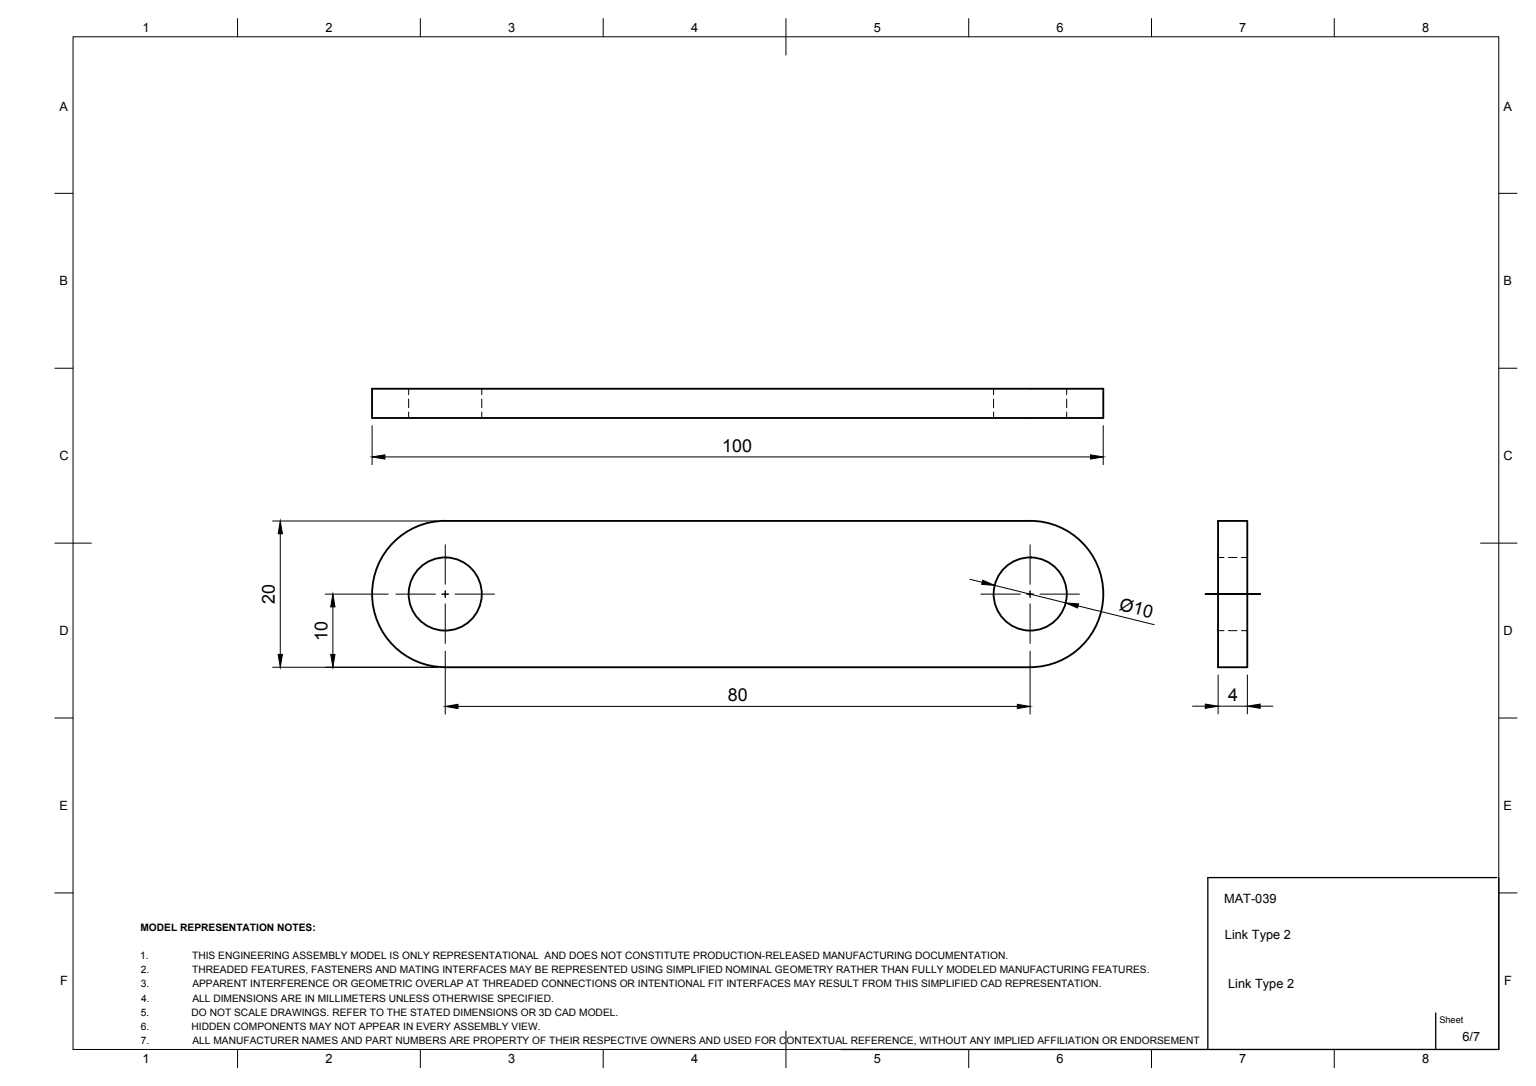
ISO-10303-21;
HEADER;
/* Generated by software containing ST-Developer
 * from STEP Tools, Inc. (www.steptools.com) 
 */

FILE_DESCRIPTION(
/* description */ ('STEP AP214'),
/* implementation_level */ '2;1');

FILE_NAME(
/* name */ 'Link Type 2.step',
/* time_stamp */ '2026-11-14T21:46:24-08:00',
/* author */ (''),
/* organization */ (''),
/* preprocessor_version */ 'ST-DEVELOPER v20.2',
/* originating_system */ 'Autodesk Translation Framework v15.17.0.0',
/* authorisation */ '');

FILE_SCHEMA (('AUTOMOTIVE_DESIGN { 1 0 10303 214 3 1 1 }'));
ENDSEC;

DATA;
#10=MECHANICAL_DESIGN_GEOMETRIC_PRESENTATION_REPRESENTATION('',(#94),#7783);
#80=SHAPE_REPRESENTATION_RELATIONSHIP('SRR','None',#7825,#87);
#87=ADVANCED_BREP_SHAPE_REPRESENTATION('',(#101),#7781);
#94=STYLED_ITEM('',(#7871),#101);
#101=MANIFOLD_SOLID_BREP('Body1',#4169);
#151=FACE_BOUND('',#1584,.T.);
#152=FACE_BOUND('',#1585,.T.);
#153=FACE_BOUND('',#1587,.T.);
#154=FACE_BOUND('',#1588,.T.);
#270=PLANE('',#4656);
#271=PLANE('',#4658);
#272=PLANE('',#4660);
#273=PLANE('',#4662);
#603=LINE('',#7614,#962);
#604=LINE('',#7620,#963);
#605=LINE('',#7627,#964);
#606=LINE('',#7630,#965);
#607=LINE('',#7633,#966);
#608=LINE('',#7636,#967);
#609=LINE('',#7639,#968);
#610=LINE('',#7642,#969);
#611=LINE('',#7644,#970);
#612=LINE('',#7646,#971);
#962=VECTOR('',#5826,5.);
#963=VECTOR('',#5833,5.);
#964=VECTOR('',#5840,1000.);
#965=VECTOR('',#5843,1000.);
#966=VECTOR('',#5846,1000.);
#967=VECTOR('',#5849,1000.);
#968=VECTOR('',#5852,1000.);
#969=VECTOR('',#5855,1000.);
#970=VECTOR('',#5858,1000.);
#971=VECTOR('',#5861,1000.);
#1078=CYLINDRICAL_SURFACE('',#4647,5.);
#1079=CYLINDRICAL_SURFACE('',#4650,5.);
#1080=CYLINDRICAL_SURFACE('',#4653,10.);
#1081=CYLINDRICAL_SURFACE('',#4661,10.);
#1298=FACE_OUTER_BOUND('',#1580,.T.);
#1299=FACE_OUTER_BOUND('',#1581,.T.);
#1300=FACE_OUTER_BOUND('',#1582,.T.);
#1301=FACE_OUTER_BOUND('',#1583,.T.);
#1302=FACE_OUTER_BOUND('',#1586,.T.);
#1303=FACE_OUTER_BOUND('',#1589,.T.);
#1304=FACE_OUTER_BOUND('',#1590,.T.);
#1305=FACE_OUTER_BOUND('',#1591,.T.);
#1580=EDGE_LOOP('',(#3768,#3769,#3770,#3771));
#1581=EDGE_LOOP('',(#3772,#3773,#3774,#3775));
#1582=EDGE_LOOP('',(#3776,#3777,#3778,#3779));
#1583=EDGE_LOOP('',(#3780,#3781,#3782,#3783));
#1584=EDGE_LOOP('',(#3784));
#1585=EDGE_LOOP('',(#3785));
#1586=EDGE_LOOP('',(#3786,#3787,#3788,#3789));
#1587=EDGE_LOOP('',(#3790));
#1588=EDGE_LOOP('',(#3791));
#1589=EDGE_LOOP('',(#3792,#3793,#3794,#3795));
#1590=EDGE_LOOP('',(#3796,#3797,#3798,#3799));
#1591=EDGE_LOOP('',(#3800,#3801,#3802,#3803));
#1800=CIRCLE('',#4648,5.);
#1801=CIRCLE('',#4649,5.);
#1802=CIRCLE('',#4651,5.);
#1803=CIRCLE('',#4652,5.);
#1804=CIRCLE('',#4654,10.);
#1805=CIRCLE('',#4655,10.);
#1806=CIRCLE('',#4657,10.);
#1807=CIRCLE('',#4659,10.);
#2142=VERTEX_POINT('',#7611);
#2143=VERTEX_POINT('',#7613);
#2144=VERTEX_POINT('',#7617);
#2145=VERTEX_POINT('',#7619);
#2146=VERTEX_POINT('',#7623);
#2147=VERTEX_POINT('',#7624);
#2148=VERTEX_POINT('',#7626);
#2149=VERTEX_POINT('',#7628);
#2150=VERTEX_POINT('',#7632);
#2151=VERTEX_POINT('',#7634);
#2152=VERTEX_POINT('',#7638);
#2153=VERTEX_POINT('',#7640);
#2691=EDGE_CURVE('',#2142,#2142,#1800,.T.);
#2692=EDGE_CURVE('',#2142,#2143,#603,.T.);
#2693=EDGE_CURVE('',#2143,#2143,#1801,.T.);
#2694=EDGE_CURVE('',#2144,#2144,#1802,.T.);
#2695=EDGE_CURVE('',#2144,#2145,#604,.T.);
#2696=EDGE_CURVE('',#2145,#2145,#1803,.T.);
#2697=EDGE_CURVE('',#2146,#2147,#1804,.T.);
#2698=EDGE_CURVE('',#2146,#2148,#605,.T.);
#2699=EDGE_CURVE('',#2148,#2149,#1805,.T.);
#2700=EDGE_CURVE('',#2147,#2149,#606,.T.);
#2701=EDGE_CURVE('',#2147,#2150,#607,.T.);
#2702=EDGE_CURVE('',#2150,#2151,#1806,.T.);
#2703=EDGE_CURVE('',#2151,#2146,#608,.T.);
#2704=EDGE_CURVE('',#2152,#2148,#609,.T.);
#2705=EDGE_CURVE('',#2153,#2152,#1807,.T.);
#2706=EDGE_CURVE('',#2149,#2153,#610,.T.);
#2707=EDGE_CURVE('',#2150,#2153,#611,.T.);
#2708=EDGE_CURVE('',#2151,#2152,#612,.T.);
#3768=ORIENTED_EDGE('',*,*,#2691,.T.);
#3769=ORIENTED_EDGE('',*,*,#2692,.T.);
#3770=ORIENTED_EDGE('',*,*,#2693,.F.);
#3771=ORIENTED_EDGE('',*,*,#2692,.F.);
#3772=ORIENTED_EDGE('',*,*,#2694,.T.);
#3773=ORIENTED_EDGE('',*,*,#2695,.T.);
#3774=ORIENTED_EDGE('',*,*,#2696,.F.);
#3775=ORIENTED_EDGE('',*,*,#2695,.F.);
#3776=ORIENTED_EDGE('',*,*,#2697,.F.);
#3777=ORIENTED_EDGE('',*,*,#2698,.T.);
#3778=ORIENTED_EDGE('',*,*,#2699,.T.);
#3779=ORIENTED_EDGE('',*,*,#2700,.F.);
#3780=ORIENTED_EDGE('',*,*,#2697,.T.);
#3781=ORIENTED_EDGE('',*,*,#2701,.T.);
#3782=ORIENTED_EDGE('',*,*,#2702,.T.);
#3783=ORIENTED_EDGE('',*,*,#2703,.T.);
#3784=ORIENTED_EDGE('',*,*,#2691,.F.);
#3785=ORIENTED_EDGE('',*,*,#2694,.F.);
#3786=ORIENTED_EDGE('',*,*,#2699,.F.);
#3787=ORIENTED_EDGE('',*,*,#2704,.F.);
#3788=ORIENTED_EDGE('',*,*,#2705,.F.);
#3789=ORIENTED_EDGE('',*,*,#2706,.F.);
#3790=ORIENTED_EDGE('',*,*,#2693,.T.);
#3791=ORIENTED_EDGE('',*,*,#2696,.T.);
#3792=ORIENTED_EDGE('',*,*,#2706,.T.);
#3793=ORIENTED_EDGE('',*,*,#2707,.F.);
#3794=ORIENTED_EDGE('',*,*,#2701,.F.);
#3795=ORIENTED_EDGE('',*,*,#2700,.T.);
#3796=ORIENTED_EDGE('',*,*,#2705,.T.);
#3797=ORIENTED_EDGE('',*,*,#2708,.F.);
#3798=ORIENTED_EDGE('',*,*,#2702,.F.);
#3799=ORIENTED_EDGE('',*,*,#2707,.T.);
#3800=ORIENTED_EDGE('',*,*,#2704,.T.);
#3801=ORIENTED_EDGE('',*,*,#2698,.F.);
#3802=ORIENTED_EDGE('',*,*,#2703,.F.);
#3803=ORIENTED_EDGE('',*,*,#2708,.T.);
#4133=ADVANCED_FACE('',(#1298),#1078,.F.);
#4134=ADVANCED_FACE('',(#1299),#1079,.F.);
#4135=ADVANCED_FACE('',(#1300),#1080,.T.);
#4136=ADVANCED_FACE('',(#1301,#151,#152),#270,.T.);
#4137=ADVANCED_FACE('',(#1302,#153,#154),#271,.F.);
#4138=ADVANCED_FACE('',(#1303),#272,.F.);
#4139=ADVANCED_FACE('',(#1304),#1081,.T.);
#4140=ADVANCED_FACE('',(#1305),#273,.F.);
#4169=CLOSED_SHELL('',(#4133,#4134,#4135,#4136,#4137,#4138,#4139,#4140));
#4646=AXIS2_PLACEMENT_3D('',#7609,#5820,#5821);
#4647=AXIS2_PLACEMENT_3D('',#7610,#5822,#5823);
#4648=AXIS2_PLACEMENT_3D('',#7612,#5824,#5825);
#4649=AXIS2_PLACEMENT_3D('',#7615,#5827,#5828);
#4650=AXIS2_PLACEMENT_3D('',#7616,#5829,#5830);
#4651=AXIS2_PLACEMENT_3D('',#7618,#5831,#5832);
#4652=AXIS2_PLACEMENT_3D('',#7621,#5834,#5835);
#4653=AXIS2_PLACEMENT_3D('',#7622,#5836,#5837);
#4654=AXIS2_PLACEMENT_3D('',#7625,#5838,#5839);
#4655=AXIS2_PLACEMENT_3D('',#7629,#5841,#5842);
#4656=AXIS2_PLACEMENT_3D('',#7631,#5844,#5845);
#4657=AXIS2_PLACEMENT_3D('',#7635,#5847,#5848);
#4658=AXIS2_PLACEMENT_3D('',#7637,#5850,#5851);
#4659=AXIS2_PLACEMENT_3D('',#7641,#5853,#5854);
#4660=AXIS2_PLACEMENT_3D('',#7643,#5856,#5857);
#4661=AXIS2_PLACEMENT_3D('',#7645,#5859,#5860);
#4662=AXIS2_PLACEMENT_3D('',#7647,#5862,#5863);
#5820=DIRECTION('axis',(0.,0.,1.));
#5821=DIRECTION('refdir',(1.,0.,0.));
#5822=DIRECTION('center_axis',(0.,0.,-1.));
#5823=DIRECTION('ref_axis',(-1.,0.,0.));
#5824=DIRECTION('center_axis',(0.,0.,1.));
#5825=DIRECTION('ref_axis',(1.,0.,0.));
#5826=DIRECTION('',(0.,0.,-1.));
#5827=DIRECTION('center_axis',(0.,0.,1.));
#5828=DIRECTION('ref_axis',(1.,0.,0.));
#5829=DIRECTION('center_axis',(0.,0.,-1.));
#5830=DIRECTION('ref_axis',(-1.,0.,0.));
#5831=DIRECTION('center_axis',(0.,0.,1.));
#5832=DIRECTION('ref_axis',(1.,0.,0.));
#5833=DIRECTION('',(0.,0.,-1.));
#5834=DIRECTION('center_axis',(0.,0.,1.));
#5835=DIRECTION('ref_axis',(1.,0.,0.));
#5836=DIRECTION('center_axis',(0.,0.,-1.));
#5837=DIRECTION('ref_axis',(-1.,0.,0.));
#5838=DIRECTION('center_axis',(0.,0.,1.));
#5839=DIRECTION('ref_axis',(1.,0.,0.));
#5840=DIRECTION('',(0.,0.,-1.));
#5841=DIRECTION('center_axis',(0.,0.,1.));
#5842=DIRECTION('ref_axis',(1.,0.,0.));
#5843=DIRECTION('',(0.,0.,-1.));
#5844=DIRECTION('center_axis',(0.,0.,1.));
#5845=DIRECTION('ref_axis',(1.,0.,0.));
#5846=DIRECTION('',(1.,1.30104260698261E-16,0.));
#5847=DIRECTION('center_axis',(0.,0.,1.));
#5848=DIRECTION('ref_axis',(-1.,0.,0.));
#5849=DIRECTION('',(-1.,0.,0.));
#5850=DIRECTION('center_axis',(0.,0.,1.));
#5851=DIRECTION('ref_axis',(1.,0.,0.));
#5852=DIRECTION('',(-1.,0.,0.));
#5853=DIRECTION('center_axis',(0.,0.,1.));
#5854=DIRECTION('ref_axis',(-1.,0.,0.));
#5855=DIRECTION('',(1.,1.30104260698261E-16,0.));
#5856=DIRECTION('center_axis',(-1.30104260698261E-16,1.,0.));
#5857=DIRECTION('ref_axis',(-1.,-1.30104260698261E-16,0.));
#5858=DIRECTION('',(0.,0.,-1.));
#5859=DIRECTION('center_axis',(0.,0.,-1.));
#5860=DIRECTION('ref_axis',(1.,1.22464679914735E-16,0.));
#5861=DIRECTION('',(0.,0.,-1.));
#5862=DIRECTION('center_axis',(0.,-1.,0.));
#5863=DIRECTION('ref_axis',(0.,0.,-1.));
#7609=CARTESIAN_POINT('',(0.,0.,0.));
#7610=CARTESIAN_POINT('Origin',(80.,6.93889390390723E-15,2.));
#7611=CARTESIAN_POINT('',(85.,6.32657050433355E-15,2.));
#7612=CARTESIAN_POINT('Origin',(80.,6.93889390390723E-15,2.));
#7613=CARTESIAN_POINT('',(85.,6.32657050433355E-15,-2.));
#7614=CARTESIAN_POINT('',(85.,6.32657050433355E-15,2.));
#7615=CARTESIAN_POINT('Origin',(80.,6.93889390390723E-15,-2.));
#7616=CARTESIAN_POINT('Origin',(0.,0.,2.));
#7617=CARTESIAN_POINT('',(5.,-6.12323399573677E-16,2.));
#7618=CARTESIAN_POINT('Origin',(0.,0.,2.));
#7619=CARTESIAN_POINT('',(5.,-6.12323399573677E-16,-2.));
#7620=CARTESIAN_POINT('',(5.,-6.12323399573677E-16,2.));
#7621=CARTESIAN_POINT('Origin',(0.,0.,-2.));
#7622=CARTESIAN_POINT('Origin',(0.,0.,2.));
#7623=CARTESIAN_POINT('',(0.,10.,2.));
#7624=CARTESIAN_POINT('',(1.22460635382238E-15,-10.,2.));
#7625=CARTESIAN_POINT('Origin',(0.,0.,2.));
#7626=CARTESIAN_POINT('',(0.,10.,-2.));
#7627=CARTESIAN_POINT('',(0.,10.,2.));
#7628=CARTESIAN_POINT('',(1.22460635382238E-15,-10.,-2.));
#7629=CARTESIAN_POINT('Origin',(0.,0.,-2.));
#7630=CARTESIAN_POINT('',(1.22460635382238E-15,-10.,2.));
#7631=CARTESIAN_POINT('Origin',(0.,0.,2.));
#7632=CARTESIAN_POINT('',(80.,-9.99999999999999,2.));
#7633=CARTESIAN_POINT('',(80.,-9.99999999999999,2.));
#7634=CARTESIAN_POINT('',(80.,10.,2.));
#7635=CARTESIAN_POINT('Origin',(80.,6.93889390390723E-15,2.));
#7636=CARTESIAN_POINT('',(0.,10.,2.));
#7637=CARTESIAN_POINT('Origin',(0.,0.,-2.));
#7638=CARTESIAN_POINT('',(80.,10.,-2.));
#7639=CARTESIAN_POINT('',(0.,10.,-2.));
#7640=CARTESIAN_POINT('',(80.,-9.99999999999999,-2.));
#7641=CARTESIAN_POINT('Origin',(80.,6.93889390390723E-15,-2.));
#7642=CARTESIAN_POINT('',(80.,-9.99999999999999,-2.));
#7643=CARTESIAN_POINT('Origin',(80.,-9.99999999999999,2.));
#7644=CARTESIAN_POINT('',(80.,-9.99999999999999,2.));
#7645=CARTESIAN_POINT('Origin',(80.,6.93889390390723E-15,2.));
#7646=CARTESIAN_POINT('',(80.,10.,2.));
#7647=CARTESIAN_POINT('Origin',(0.,10.,2.));
#7771=UNCERTAINTY_MEASURE_WITH_UNIT(LENGTH_MEASURE(0.01),#7784,
'DISTANCE_ACCURACY_VALUE',
'Maximum model space distance between geometric entities at asserted c
onnectivities');
#7773=UNCERTAINTY_MEASURE_WITH_UNIT(LENGTH_MEASURE(0.01),#7784,
'DISTANCE_ACCURACY_VALUE',
'Maximum model space distance between geometric entities at asserted c
onnectivities');
#7781=(
GEOMETRIC_REPRESENTATION_CONTEXT(3)
GLOBAL_UNCERTAINTY_ASSIGNED_CONTEXT((#7771))
GLOBAL_UNIT_ASSIGNED_CONTEXT((#7784,#7786,#7787))
REPRESENTATION_CONTEXT('','3D')
);
#7783=(
GEOMETRIC_REPRESENTATION_CONTEXT(3)
GLOBAL_UNCERTAINTY_ASSIGNED_CONTEXT((#7773))
GLOBAL_UNIT_ASSIGNED_CONTEXT((#7784,#7786,#7787))
REPRESENTATION_CONTEXT('','3D')
);
#7784=(
LENGTH_UNIT()
NAMED_UNIT(*)
SI_UNIT(.MILLI.,.METRE.)
);
#7786=(
NAMED_UNIT(*)
PLANE_ANGLE_UNIT()
SI_UNIT($,.RADIAN.)
);
#7787=(
NAMED_UNIT(*)
SI_UNIT($,.STERADIAN.)
SOLID_ANGLE_UNIT()
);
#7795=SHAPE_DEFINITION_REPRESENTATION(#7805,#7825);
#7805=PRODUCT_DEFINITION_SHAPE('',$,#7835);
#7825=SHAPE_REPRESENTATION('',(#4646),#7781);
#7827=PRODUCT_DEFINITION_CONTEXT('part definition',#7856,'design');
#7835=PRODUCT_DEFINITION('Link Type 2','Link Type 2',#7844,#7827);
#7844=PRODUCT_DEFINITION_FORMATION('',$,#7865);
#7856=APPLICATION_CONTEXT(
'Core Data for Automotive Mechanical Design Process');
#7857=PRODUCT_CONTEXT('part definition',#7856,'mechanical');
#7865=PRODUCT('Link Type 2','Link Type 2',$,(#7857));
#7871=PRESENTATION_STYLE_ASSIGNMENT((#7876));
#7876=SURFACE_STYLE_USAGE(.BOTH.,#7881);
#7881=SURFACE_SIDE_STYLE('',(#7886));
#7886=SURFACE_STYLE_FILL_AREA(#7891);
#7891=FILL_AREA_STYLE('Opaque(227,224,212)',(#7896));
#7896=FILL_AREA_STYLE_COLOUR('Opaque(227,224,212)',#7901);
#7901=COLOUR_RGB('Opaque(227,224,212)',0.890196078431372,0.87843137254902,
0.831372549019608);
ENDSEC;
END-ISO-10303-21;
